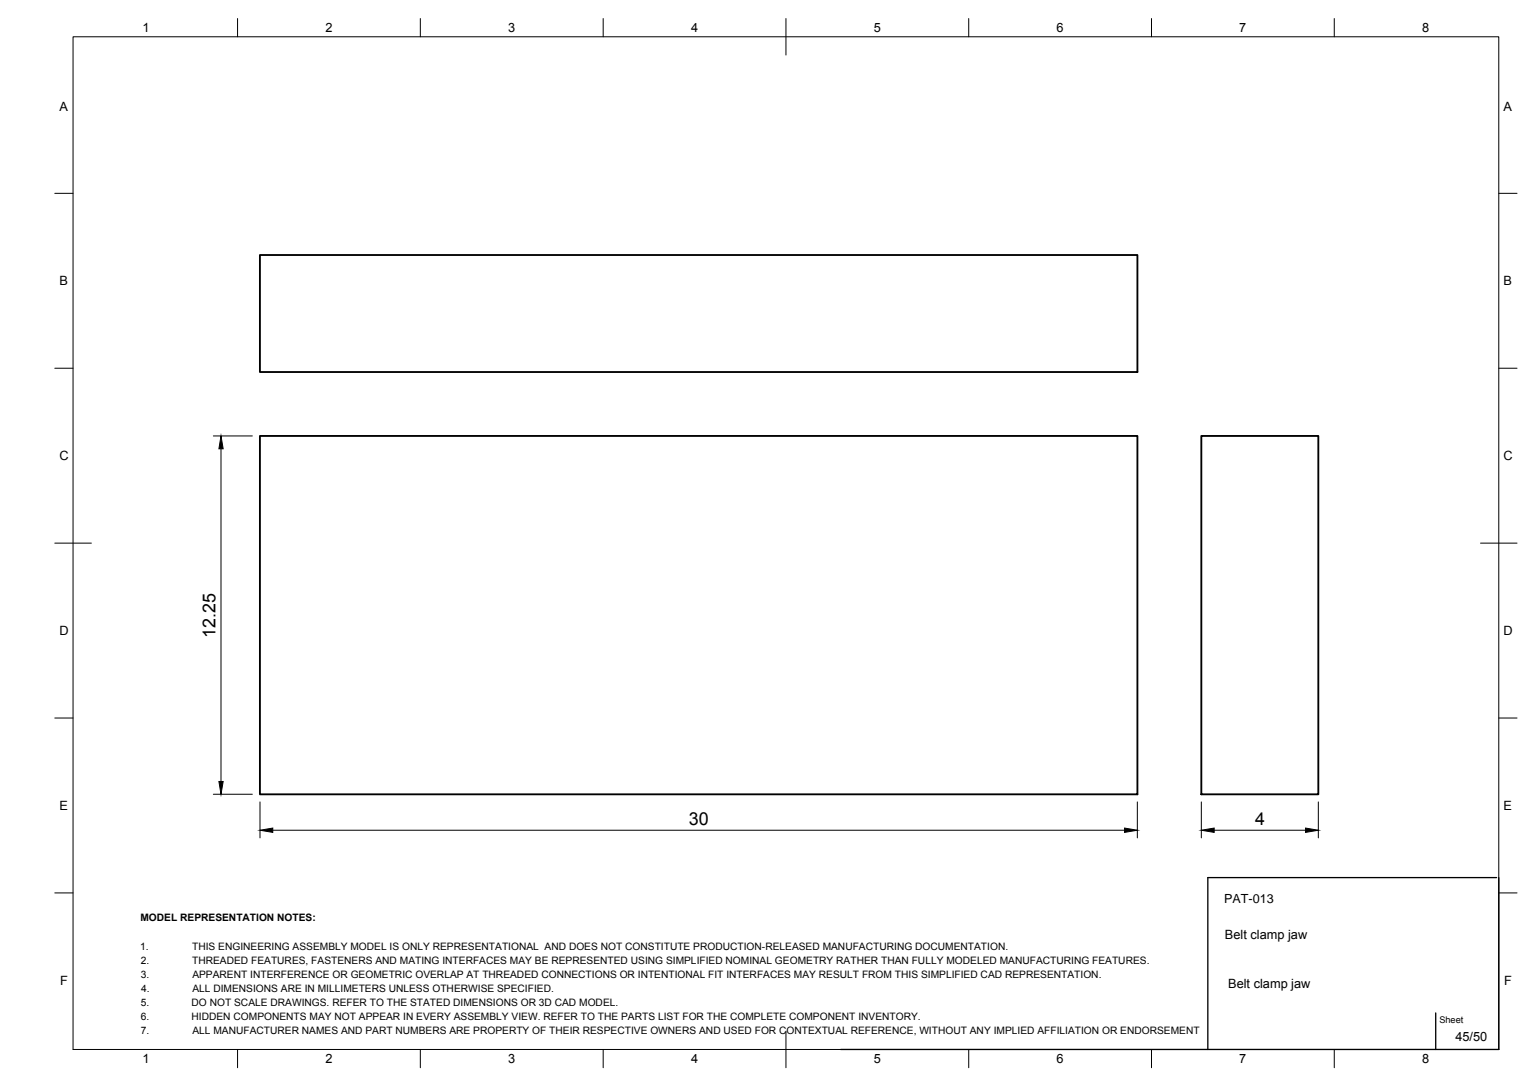
ISO-10303-21;
HEADER;
/* Generated by software containing ST-Developer
 * from STEP Tools, Inc. (www.steptools.com) 
 */

FILE_DESCRIPTION(
/* description */ ('Belt-driven linear axis on 2020 extrusion'),
/* implementation_level */ '2;1');

FILE_NAME(
/* name */ 'Belt clamp jaw.step',
/* time_stamp */ '2026-10-28T03:26:09-07:00',
/* author */ (''),
/* organization */ (''),
/* preprocessor_version */ 'ST-DEVELOPER v20.2',
/* originating_system */ 'Autodesk Translation Framework v15.17.0.0',
/* authorisation */ '');

FILE_SCHEMA (('AUTOMOTIVE_DESIGN { 1 0 10303 214 3 1 1 }'));
ENDSEC;

DATA;
#10=MECHANICAL_DESIGN_GEOMETRIC_PRESENTATION_REPRESENTATION('',(#658),#20096);
#556=SHAPE_REPRESENTATION_RELATIONSHIP('SRR','None',#20356,#602);
#602=ADVANCED_BREP_SHAPE_REPRESENTATION('',(#713),#20087);
#658=STYLED_ITEM('',(#20657),#713);
#713=MANIFOLD_SOLID_BREP('Body1',#10972);
#1171=PLANE('',#12530);
#1172=PLANE('',#12531);
#1173=PLANE('',#12532);
#1174=PLANE('',#12533);
#1175=PLANE('',#12534);
#1176=PLANE('',#12535);
#1769=FACE_OUTER_BOUND('',#2553,.T.);
#1770=FACE_OUTER_BOUND('',#2554,.T.);
#1771=FACE_OUTER_BOUND('',#2555,.T.);
#1772=FACE_OUTER_BOUND('',#2556,.T.);
#1773=FACE_OUTER_BOUND('',#2557,.T.);
#1774=FACE_OUTER_BOUND('',#2558,.T.);
#2553=EDGE_LOOP('',(#9609,#9610,#9611,#9612));
#2554=EDGE_LOOP('',(#9613,#9614,#9615,#9616));
#2555=EDGE_LOOP('',(#9617,#9618,#9619,#9620));
#2556=EDGE_LOOP('',(#9621,#9622,#9623,#9624));
#2557=EDGE_LOOP('',(#9625,#9626,#9627,#9628));
#2558=EDGE_LOOP('',(#9629,#9630,#9631,#9632));
#3332=LINE('',#19395,#4189);
#3333=LINE('',#19397,#4190);
#3334=LINE('',#19399,#4191);
#3335=LINE('',#19400,#4192);
#3336=LINE('',#19403,#4193);
#3337=LINE('',#19405,#4194);
#3338=LINE('',#19406,#4195);
#3339=LINE('',#19409,#4196);
#3340=LINE('',#19411,#4197);
#3341=LINE('',#19412,#4198);
#3342=LINE('',#19414,#4199);
#3343=LINE('',#19415,#4200);
#4189=VECTOR('',#15534,1.);
#4190=VECTOR('',#15535,1.);
#4191=VECTOR('',#15536,1.);
#4192=VECTOR('',#15537,1.);
#4193=VECTOR('',#15540,1.);
#4194=VECTOR('',#15541,1.);
#4195=VECTOR('',#15542,1.);
#4196=VECTOR('',#15545,1.);
#4197=VECTOR('',#15546,1.);
#4198=VECTOR('',#15547,1.);
#4199=VECTOR('',#15550,1.);
#4200=VECTOR('',#15551,1.);
#5689=VERTEX_POINT('',#19393);
#5690=VERTEX_POINT('',#19394);
#5691=VERTEX_POINT('',#19396);
#5692=VERTEX_POINT('',#19398);
#5693=VERTEX_POINT('',#19402);
#5694=VERTEX_POINT('',#19404);
#5695=VERTEX_POINT('',#19408);
#5696=VERTEX_POINT('',#19410);
#7019=EDGE_CURVE('',#5689,#5690,#3332,.T.);
#7020=EDGE_CURVE('',#5690,#5691,#3333,.T.);
#7021=EDGE_CURVE('',#5692,#5691,#3334,.T.);
#7022=EDGE_CURVE('',#5689,#5692,#3335,.T.);
#7023=EDGE_CURVE('',#5693,#5689,#3336,.T.);
#7024=EDGE_CURVE('',#5694,#5692,#3337,.T.);
#7025=EDGE_CURVE('',#5693,#5694,#3338,.T.);
#7026=EDGE_CURVE('',#5695,#5693,#3339,.T.);
#7027=EDGE_CURVE('',#5696,#5694,#3340,.T.);
#7028=EDGE_CURVE('',#5695,#5696,#3341,.T.);
#7029=EDGE_CURVE('',#5690,#5695,#3342,.T.);
#7030=EDGE_CURVE('',#5691,#5696,#3343,.T.);
#9609=ORIENTED_EDGE('',*,*,#7019,.T.);
#9610=ORIENTED_EDGE('',*,*,#7020,.T.);
#9611=ORIENTED_EDGE('',*,*,#7021,.F.);
#9612=ORIENTED_EDGE('',*,*,#7022,.F.);
#9613=ORIENTED_EDGE('',*,*,#7023,.T.);
#9614=ORIENTED_EDGE('',*,*,#7022,.T.);
#9615=ORIENTED_EDGE('',*,*,#7024,.F.);
#9616=ORIENTED_EDGE('',*,*,#7025,.F.);
#9617=ORIENTED_EDGE('',*,*,#7026,.T.);
#9618=ORIENTED_EDGE('',*,*,#7025,.T.);
#9619=ORIENTED_EDGE('',*,*,#7027,.F.);
#9620=ORIENTED_EDGE('',*,*,#7028,.F.);
#9621=ORIENTED_EDGE('',*,*,#7029,.T.);
#9622=ORIENTED_EDGE('',*,*,#7028,.T.);
#9623=ORIENTED_EDGE('',*,*,#7030,.F.);
#9624=ORIENTED_EDGE('',*,*,#7020,.F.);
#9625=ORIENTED_EDGE('',*,*,#7030,.T.);
#9626=ORIENTED_EDGE('',*,*,#7027,.T.);
#9627=ORIENTED_EDGE('',*,*,#7024,.T.);
#9628=ORIENTED_EDGE('',*,*,#7021,.T.);
#9629=ORIENTED_EDGE('',*,*,#7029,.F.);
#9630=ORIENTED_EDGE('',*,*,#7019,.F.);
#9631=ORIENTED_EDGE('',*,*,#7023,.F.);
#9632=ORIENTED_EDGE('',*,*,#7026,.F.);
#10820=ADVANCED_FACE('',(#1769),#1171,.T.);
#10821=ADVANCED_FACE('',(#1770),#1172,.T.);
#10822=ADVANCED_FACE('',(#1771),#1173,.T.);
#10823=ADVANCED_FACE('',(#1772),#1174,.T.);
#10824=ADVANCED_FACE('',(#1773),#1175,.T.);
#10825=ADVANCED_FACE('',(#1774),#1176,.F.);
#10972=CLOSED_SHELL('',(#10820,#10821,#10822,#10823,#10824,#10825));
#12529=AXIS2_PLACEMENT_3D('',#19391,#15530,#15531);
#12530=AXIS2_PLACEMENT_3D('',#19392,#15532,#15533);
#12531=AXIS2_PLACEMENT_3D('',#19401,#15538,#15539);
#12532=AXIS2_PLACEMENT_3D('',#19407,#15543,#15544);
#12533=AXIS2_PLACEMENT_3D('',#19413,#15548,#15549);
#12534=AXIS2_PLACEMENT_3D('',#19416,#15552,#15553);
#12535=AXIS2_PLACEMENT_3D('',#19417,#15554,#15555);
#15530=DIRECTION('axis',(0.,0.,1.));
#15531=DIRECTION('refdir',(1.,0.,0.));
#15532=DIRECTION('center_axis',(0.,1.,0.));
#15533=DIRECTION('ref_axis',(-1.,0.,0.));
#15534=DIRECTION('',(-1.,0.,0.));
#15535=DIRECTION('',(0.,0.,1.));
#15536=DIRECTION('',(-1.,0.,0.));
#15537=DIRECTION('',(0.,0.,1.));
#15538=DIRECTION('center_axis',(1.,0.,0.));
#15539=DIRECTION('ref_axis',(0.,1.,0.));
#15540=DIRECTION('',(0.,1.,0.));
#15541=DIRECTION('',(0.,1.,0.));
#15542=DIRECTION('',(0.,0.,1.));
#15543=DIRECTION('center_axis',(0.,-1.,0.));
#15544=DIRECTION('ref_axis',(1.,0.,0.));
#15545=DIRECTION('',(1.,0.,0.));
#15546=DIRECTION('',(1.,0.,0.));
#15547=DIRECTION('',(0.,0.,1.));
#15548=DIRECTION('center_axis',(-1.,0.,0.));
#15549=DIRECTION('ref_axis',(0.,-1.,0.));
#15550=DIRECTION('',(0.,-1.,0.));
#15551=DIRECTION('',(0.,-1.,0.));
#15552=DIRECTION('center_axis',(0.,0.,1.));
#15553=DIRECTION('ref_axis',(1.,0.,0.));
#15554=DIRECTION('center_axis',(0.,0.,1.));
#15555=DIRECTION('ref_axis',(1.,0.,0.));
#19391=CARTESIAN_POINT('',(0.,0.,0.));
#19392=CARTESIAN_POINT('Origin',(17.5,-2.2,7.23661977));
#19393=CARTESIAN_POINT('',(17.5,-2.2,7.23661977));
#19394=CARTESIAN_POINT('',(14.5,-2.2,7.23661977));
#19395=CARTESIAN_POINT('',(17.5,-2.2,7.23661977));
#19396=CARTESIAN_POINT('',(14.5,-2.2,7.63661977));
#19397=CARTESIAN_POINT('',(14.5,-2.2,7.23661977));
#19398=CARTESIAN_POINT('',(17.5,-2.2,7.63661977));
#19399=CARTESIAN_POINT('',(17.5,-2.2,7.63661977));
#19400=CARTESIAN_POINT('',(17.5,-2.2,7.23661977));
#19401=CARTESIAN_POINT('Origin',(17.5,-3.425,7.23661977));
#19402=CARTESIAN_POINT('',(17.5,-3.425,7.23661977));
#19403=CARTESIAN_POINT('',(17.5,-3.425,7.23661977));
#19404=CARTESIAN_POINT('',(17.5,-3.425,7.63661977));
#19405=CARTESIAN_POINT('',(17.5,-3.425,7.63661977));
#19406=CARTESIAN_POINT('',(17.5,-3.425,7.23661977));
#19407=CARTESIAN_POINT('Origin',(14.5,-3.425,7.23661977));
#19408=CARTESIAN_POINT('',(14.5,-3.425,7.23661977));
#19409=CARTESIAN_POINT('',(14.5,-3.425,7.23661977));
#19410=CARTESIAN_POINT('',(14.5,-3.425,7.63661977));
#19411=CARTESIAN_POINT('',(14.5,-3.425,7.63661977));
#19412=CARTESIAN_POINT('',(14.5,-3.425,7.23661977));
#19413=CARTESIAN_POINT('Origin',(14.5,-2.2,7.23661977));
#19414=CARTESIAN_POINT('',(14.5,-2.2,7.23661977));
#19415=CARTESIAN_POINT('',(14.5,-2.2,7.63661977));
#19416=CARTESIAN_POINT('Origin',(16.,-2.8125,7.63661977));
#19417=CARTESIAN_POINT('Origin',(16.,-2.8125,7.23661977));
#20033=UNCERTAINTY_MEASURE_WITH_UNIT(LENGTH_MEASURE(0.001),#20097,
'DISTANCE_ACCURACY_VALUE',
'Maximum model space distance between geometric entities at asserted c
onnectivities');
#20042=UNCERTAINTY_MEASURE_WITH_UNIT(LENGTH_MEASURE(0.001),#20097,
'DISTANCE_ACCURACY_VALUE',
'Maximum model space distance between geometric entities at asserted c
onnectivities');
#20087=(
GEOMETRIC_REPRESENTATION_CONTEXT(3)
GLOBAL_UNCERTAINTY_ASSIGNED_CONTEXT((#20033))
GLOBAL_UNIT_ASSIGNED_CONTEXT((#20097,#20099,#20100))
REPRESENTATION_CONTEXT('','3D')
);
#20096=(
GEOMETRIC_REPRESENTATION_CONTEXT(3)
GLOBAL_UNCERTAINTY_ASSIGNED_CONTEXT((#20042))
GLOBAL_UNIT_ASSIGNED_CONTEXT((#20097,#20099,#20100))
REPRESENTATION_CONTEXT('','3D')
);
#20097=(
LENGTH_UNIT()
NAMED_UNIT(*)
SI_UNIT(.CENTI.,.METRE.)
);
#20099=(
NAMED_UNIT(*)
PLANE_ANGLE_UNIT()
SI_UNIT($,.RADIAN.)
);
#20100=(
NAMED_UNIT(*)
SI_UNIT($,.STERADIAN.)
SOLID_ANGLE_UNIT()
);
#20145=SHAPE_DEFINITION_REPRESENTATION(#20203,#20356);
#20203=PRODUCT_DEFINITION_SHAPE('',$,#20410);
#20356=SHAPE_REPRESENTATION('',(#12529),#20087);
#20365=PRODUCT_DEFINITION_CONTEXT('part definition',#20526,'design');
#20410=PRODUCT_DEFINITION('Belt clamp jaw','Belt clamp jaw',#20463,#20365);
#20463=PRODUCT_DEFINITION_FORMATION('',$,#20572);
#20526=APPLICATION_CONTEXT(
'Core Data for Automotive Mechanical Design Process');
#20527=PRODUCT_CONTEXT('part definition',#20526,'mechanical');
#20572=PRODUCT('Belt clamp jaw','Belt clamp jaw','Belt clamp jaw',(#20527));
#20651=COLOUR_RGB('Black',0.12,0.14,0.17);
#20652=FILL_AREA_STYLE_COLOUR('',#20651);
#20653=FILL_AREA_STYLE('',(#20652));
#20654=SURFACE_STYLE_FILL_AREA(#20653);
#20655=SURFACE_SIDE_STYLE('',(#20654));
#20656=SURFACE_STYLE_USAGE(.BOTH.,#20655);
#20657=PRESENTATION_STYLE_ASSIGNMENT((#20656));
ENDSEC;
END-ISO-10303-21;
